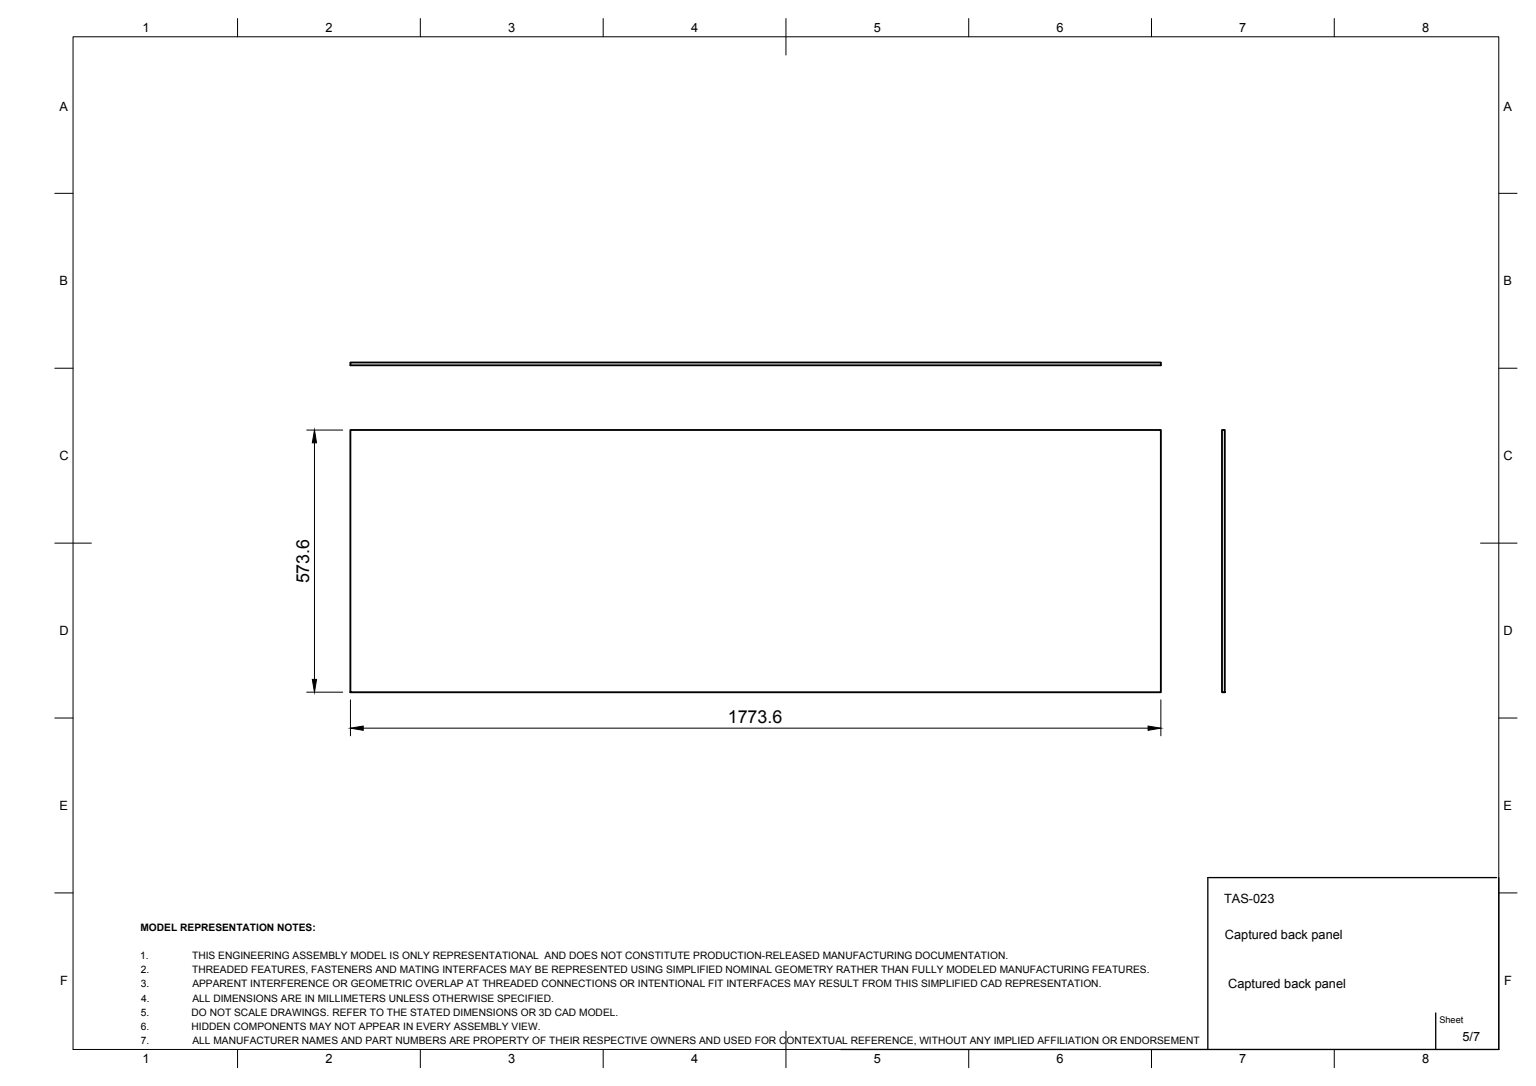
ISO-10303-21;
HEADER;
/* Generated by software containing ST-Developer
 * from STEP Tools, Inc. (www.steptools.com) 
 */

FILE_DESCRIPTION(
/* description */ (''),
/* implementation_level */ '2;1');

FILE_NAME(
/* name */ 'Captured back panel.step',
/* time_stamp */ '2026-11-15T17:51:54-08:00',
/* author */ (''),
/* organization */ (''),
/* preprocessor_version */ 'ST-DEVELOPER v20.2',
/* originating_system */ 'Autodesk Translation Framework v15.17.0.0',
/* authorisation */ '');

FILE_SCHEMA (('AUTOMOTIVE_DESIGN { 1 0 10303 214 3 1 1 }'));
ENDSEC;

DATA;
#10=MECHANICAL_DESIGN_GEOMETRIC_PRESENTATION_REPRESENTATION('',(#119),#2860);
#109=SHAPE_REPRESENTATION_RELATIONSHIP('SRR','None',#2904,#114);
#114=ADVANCED_BREP_SHAPE_REPRESENTATION('',(#124),#2857);
#119=STYLED_ITEM('',(#2938),#124);
#124=MANIFOLD_SOLID_BREP('Body1',#1716);
#199=PLANE('',#1859);
#200=PLANE('',#1860);
#201=PLANE('',#1861);
#202=PLANE('',#1862);
#203=PLANE('',#1863);
#204=PLANE('',#1864);
#285=FACE_OUTER_BOUND('',#376,.T.);
#286=FACE_OUTER_BOUND('',#377,.T.);
#287=FACE_OUTER_BOUND('',#378,.T.);
#288=FACE_OUTER_BOUND('',#379,.T.);
#289=FACE_OUTER_BOUND('',#380,.T.);
#290=FACE_OUTER_BOUND('',#381,.T.);
#376=EDGE_LOOP('',(#1568,#1569,#1570,#1571));
#377=EDGE_LOOP('',(#1572,#1573,#1574,#1575));
#378=EDGE_LOOP('',(#1576,#1577,#1578,#1579));
#379=EDGE_LOOP('',(#1580,#1581,#1582,#1583));
#380=EDGE_LOOP('',(#1584,#1585,#1586,#1587));
#381=EDGE_LOOP('',(#1588,#1589,#1590,#1591));
#575=LINE('',#2764,#784);
#576=LINE('',#2766,#785);
#577=LINE('',#2768,#786);
#578=LINE('',#2769,#787);
#579=LINE('',#2772,#788);
#580=LINE('',#2774,#789);
#581=LINE('',#2775,#790);
#582=LINE('',#2778,#791);
#583=LINE('',#2780,#792);
#584=LINE('',#2781,#793);
#585=LINE('',#2783,#794);
#586=LINE('',#2784,#795);
#784=VECTOR('',#2256,1.);
#785=VECTOR('',#2257,1.);
#786=VECTOR('',#2258,1.);
#787=VECTOR('',#2259,1.);
#788=VECTOR('',#2262,1.);
#789=VECTOR('',#2263,1.);
#790=VECTOR('',#2264,1.);
#791=VECTOR('',#2267,1.);
#792=VECTOR('',#2268,1.);
#793=VECTOR('',#2269,1.);
#794=VECTOR('',#2272,1.);
#795=VECTOR('',#2273,1.);
#947=VERTEX_POINT('',#2762);
#948=VERTEX_POINT('',#2763);
#949=VERTEX_POINT('',#2765);
#950=VERTEX_POINT('',#2767);
#951=VERTEX_POINT('',#2771);
#952=VERTEX_POINT('',#2773);
#953=VERTEX_POINT('',#2777);
#954=VERTEX_POINT('',#2779);
#1157=EDGE_CURVE('',#947,#948,#575,.T.);
#1158=EDGE_CURVE('',#948,#949,#576,.T.);
#1159=EDGE_CURVE('',#950,#949,#577,.T.);
#1160=EDGE_CURVE('',#947,#950,#578,.T.);
#1161=EDGE_CURVE('',#951,#947,#579,.T.);
#1162=EDGE_CURVE('',#952,#950,#580,.T.);
#1163=EDGE_CURVE('',#951,#952,#581,.T.);
#1164=EDGE_CURVE('',#953,#951,#582,.T.);
#1165=EDGE_CURVE('',#954,#952,#583,.T.);
#1166=EDGE_CURVE('',#953,#954,#584,.T.);
#1167=EDGE_CURVE('',#948,#953,#585,.T.);
#1168=EDGE_CURVE('',#949,#954,#586,.T.);
#1568=ORIENTED_EDGE('',*,*,#1157,.T.);
#1569=ORIENTED_EDGE('',*,*,#1158,.T.);
#1570=ORIENTED_EDGE('',*,*,#1159,.F.);
#1571=ORIENTED_EDGE('',*,*,#1160,.F.);
#1572=ORIENTED_EDGE('',*,*,#1161,.T.);
#1573=ORIENTED_EDGE('',*,*,#1160,.T.);
#1574=ORIENTED_EDGE('',*,*,#1162,.F.);
#1575=ORIENTED_EDGE('',*,*,#1163,.F.);
#1576=ORIENTED_EDGE('',*,*,#1164,.T.);
#1577=ORIENTED_EDGE('',*,*,#1163,.T.);
#1578=ORIENTED_EDGE('',*,*,#1165,.F.);
#1579=ORIENTED_EDGE('',*,*,#1166,.F.);
#1580=ORIENTED_EDGE('',*,*,#1167,.T.);
#1581=ORIENTED_EDGE('',*,*,#1166,.T.);
#1582=ORIENTED_EDGE('',*,*,#1168,.F.);
#1583=ORIENTED_EDGE('',*,*,#1158,.F.);
#1584=ORIENTED_EDGE('',*,*,#1168,.T.);
#1585=ORIENTED_EDGE('',*,*,#1165,.T.);
#1586=ORIENTED_EDGE('',*,*,#1162,.T.);
#1587=ORIENTED_EDGE('',*,*,#1159,.T.);
#1588=ORIENTED_EDGE('',*,*,#1167,.F.);
#1589=ORIENTED_EDGE('',*,*,#1157,.F.);
#1590=ORIENTED_EDGE('',*,*,#1161,.F.);
#1591=ORIENTED_EDGE('',*,*,#1164,.F.);
#1699=ADVANCED_FACE('',(#285),#199,.T.);
#1700=ADVANCED_FACE('',(#286),#200,.T.);
#1701=ADVANCED_FACE('',(#287),#201,.T.);
#1702=ADVANCED_FACE('',(#288),#202,.T.);
#1703=ADVANCED_FACE('',(#289),#203,.T.);
#1704=ADVANCED_FACE('',(#290),#204,.F.);
#1716=CLOSED_SHELL('',(#1699,#1700,#1701,#1702,#1703,#1704));
#1858=AXIS2_PLACEMENT_3D('',#2760,#2252,#2253);
#1859=AXIS2_PLACEMENT_3D('',#2761,#2254,#2255);
#1860=AXIS2_PLACEMENT_3D('',#2770,#2260,#2261);
#1861=AXIS2_PLACEMENT_3D('',#2776,#2265,#2266);
#1862=AXIS2_PLACEMENT_3D('',#2782,#2270,#2271);
#1863=AXIS2_PLACEMENT_3D('',#2785,#2274,#2275);
#1864=AXIS2_PLACEMENT_3D('',#2786,#2276,#2277);
#2252=DIRECTION('axis',(0.,0.,1.));
#2253=DIRECTION('refdir',(1.,0.,0.));
#2254=DIRECTION('center_axis',(0.,1.,0.));
#2255=DIRECTION('ref_axis',(-1.,0.,0.));
#2256=DIRECTION('',(-1.,0.,0.));
#2257=DIRECTION('',(0.,0.,1.));
#2258=DIRECTION('',(-1.,0.,0.));
#2259=DIRECTION('',(0.,0.,1.));
#2260=DIRECTION('center_axis',(1.,0.,0.));
#2261=DIRECTION('ref_axis',(0.,1.,0.));
#2262=DIRECTION('',(0.,1.,0.));
#2263=DIRECTION('',(0.,1.,0.));
#2264=DIRECTION('',(0.,0.,1.));
#2265=DIRECTION('center_axis',(0.,-1.,0.));
#2266=DIRECTION('ref_axis',(1.,0.,0.));
#2267=DIRECTION('',(1.,0.,0.));
#2268=DIRECTION('',(1.,0.,0.));
#2269=DIRECTION('',(0.,0.,1.));
#2270=DIRECTION('center_axis',(-1.,0.,0.));
#2271=DIRECTION('ref_axis',(0.,-1.,0.));
#2272=DIRECTION('',(0.,-1.,0.));
#2273=DIRECTION('',(0.,-1.,0.));
#2274=DIRECTION('center_axis',(0.,0.,1.));
#2275=DIRECTION('ref_axis',(1.,0.,0.));
#2276=DIRECTION('center_axis',(0.,0.,1.));
#2277=DIRECTION('ref_axis',(1.,0.,0.));
#2760=CARTESIAN_POINT('',(0.,0.,0.));
#2761=CARTESIAN_POINT('Origin',(57.36,0.6,0.));
#2762=CARTESIAN_POINT('',(57.36,0.6,0.));
#2763=CARTESIAN_POINT('',(0.,0.6,0.));
#2764=CARTESIAN_POINT('',(57.36,0.6,0.));
#2765=CARTESIAN_POINT('',(0.,0.6,177.36));
#2766=CARTESIAN_POINT('',(0.,0.6,0.));
#2767=CARTESIAN_POINT('',(57.36,0.6,177.36));
#2768=CARTESIAN_POINT('',(57.36,0.6,177.36));
#2769=CARTESIAN_POINT('',(57.36,0.6,0.));
#2770=CARTESIAN_POINT('Origin',(57.36,0.,0.));
#2771=CARTESIAN_POINT('',(57.36,0.,0.));
#2772=CARTESIAN_POINT('',(57.36,0.,0.));
#2773=CARTESIAN_POINT('',(57.36,0.,177.36));
#2774=CARTESIAN_POINT('',(57.36,0.,177.36));
#2775=CARTESIAN_POINT('',(57.36,0.,0.));
#2776=CARTESIAN_POINT('Origin',(0.,0.,0.));
#2777=CARTESIAN_POINT('',(0.,0.,0.));
#2778=CARTESIAN_POINT('',(0.,0.,0.));
#2779=CARTESIAN_POINT('',(0.,0.,177.36));
#2780=CARTESIAN_POINT('',(0.,0.,177.36));
#2781=CARTESIAN_POINT('',(0.,0.,0.));
#2782=CARTESIAN_POINT('Origin',(0.,0.6,0.));
#2783=CARTESIAN_POINT('',(0.,0.6,0.));
#2784=CARTESIAN_POINT('',(0.,0.6,177.36));
#2785=CARTESIAN_POINT('Origin',(28.68,0.3,177.36));
#2786=CARTESIAN_POINT('Origin',(28.68,0.3,0.));
#2850=UNCERTAINTY_MEASURE_WITH_UNIT(LENGTH_MEASURE(0.001),#2861,
'DISTANCE_ACCURACY_VALUE',
'Maximum model space distance between geometric entities at asserted c
onnectivities');
#2853=UNCERTAINTY_MEASURE_WITH_UNIT(LENGTH_MEASURE(0.001),#2861,
'DISTANCE_ACCURACY_VALUE',
'Maximum model space distance between geometric entities at asserted c
onnectivities');
#2857=(
GEOMETRIC_REPRESENTATION_CONTEXT(3)
GLOBAL_UNCERTAINTY_ASSIGNED_CONTEXT((#2850))
GLOBAL_UNIT_ASSIGNED_CONTEXT((#2861,#2863,#2864))
REPRESENTATION_CONTEXT('','3D')
);
#2860=(
GEOMETRIC_REPRESENTATION_CONTEXT(3)
GLOBAL_UNCERTAINTY_ASSIGNED_CONTEXT((#2853))
GLOBAL_UNIT_ASSIGNED_CONTEXT((#2861,#2863,#2864))
REPRESENTATION_CONTEXT('','3D')
);
#2861=(
LENGTH_UNIT()
NAMED_UNIT(*)
SI_UNIT(.CENTI.,.METRE.)
);
#2863=(
NAMED_UNIT(*)
PLANE_ANGLE_UNIT()
SI_UNIT($,.RADIAN.)
);
#2864=(
NAMED_UNIT(*)
SI_UNIT($,.STERADIAN.)
SOLID_ANGLE_UNIT()
);
#2868=SHAPE_DEFINITION_REPRESENTATION(#2874,#2904);
#2874=PRODUCT_DEFINITION_SHAPE('',$,#2911);
#2904=SHAPE_REPRESENTATION('',(#1858),#2857);
#2907=PRODUCT_DEFINITION_CONTEXT('part definition',#2927,'design');
#2911=PRODUCT_DEFINITION('Captured back panel','Captured back panel',#2917,
#2907);
#2917=PRODUCT_DEFINITION_FORMATION('',$,#2932);
#2927=APPLICATION_CONTEXT(
'Core Data for Automotive Mechanical Design Process');
#2928=PRODUCT_CONTEXT('part definition',#2927,'mechanical');
#2932=PRODUCT('Captured back panel','Captured back panel',$,(#2928));
#2938=PRESENTATION_STYLE_ASSIGNMENT((#2944));
#2944=SURFACE_STYLE_USAGE(.BOTH.,#2950);
#2950=SURFACE_SIDE_STYLE('',(#2956));
#2956=SURFACE_STYLE_FILL_AREA(#2962);
#2962=FILL_AREA_STYLE('Captured back panel finish',(#2968));
#2968=FILL_AREA_STYLE_COLOUR('Captured back panel finish',#2974);
#2974=COLOUR_RGB('Captured back panel finish',0.607843137254902,0.647058823529412,
0.701960784313725);
ENDSEC;
END-ISO-10303-21;
